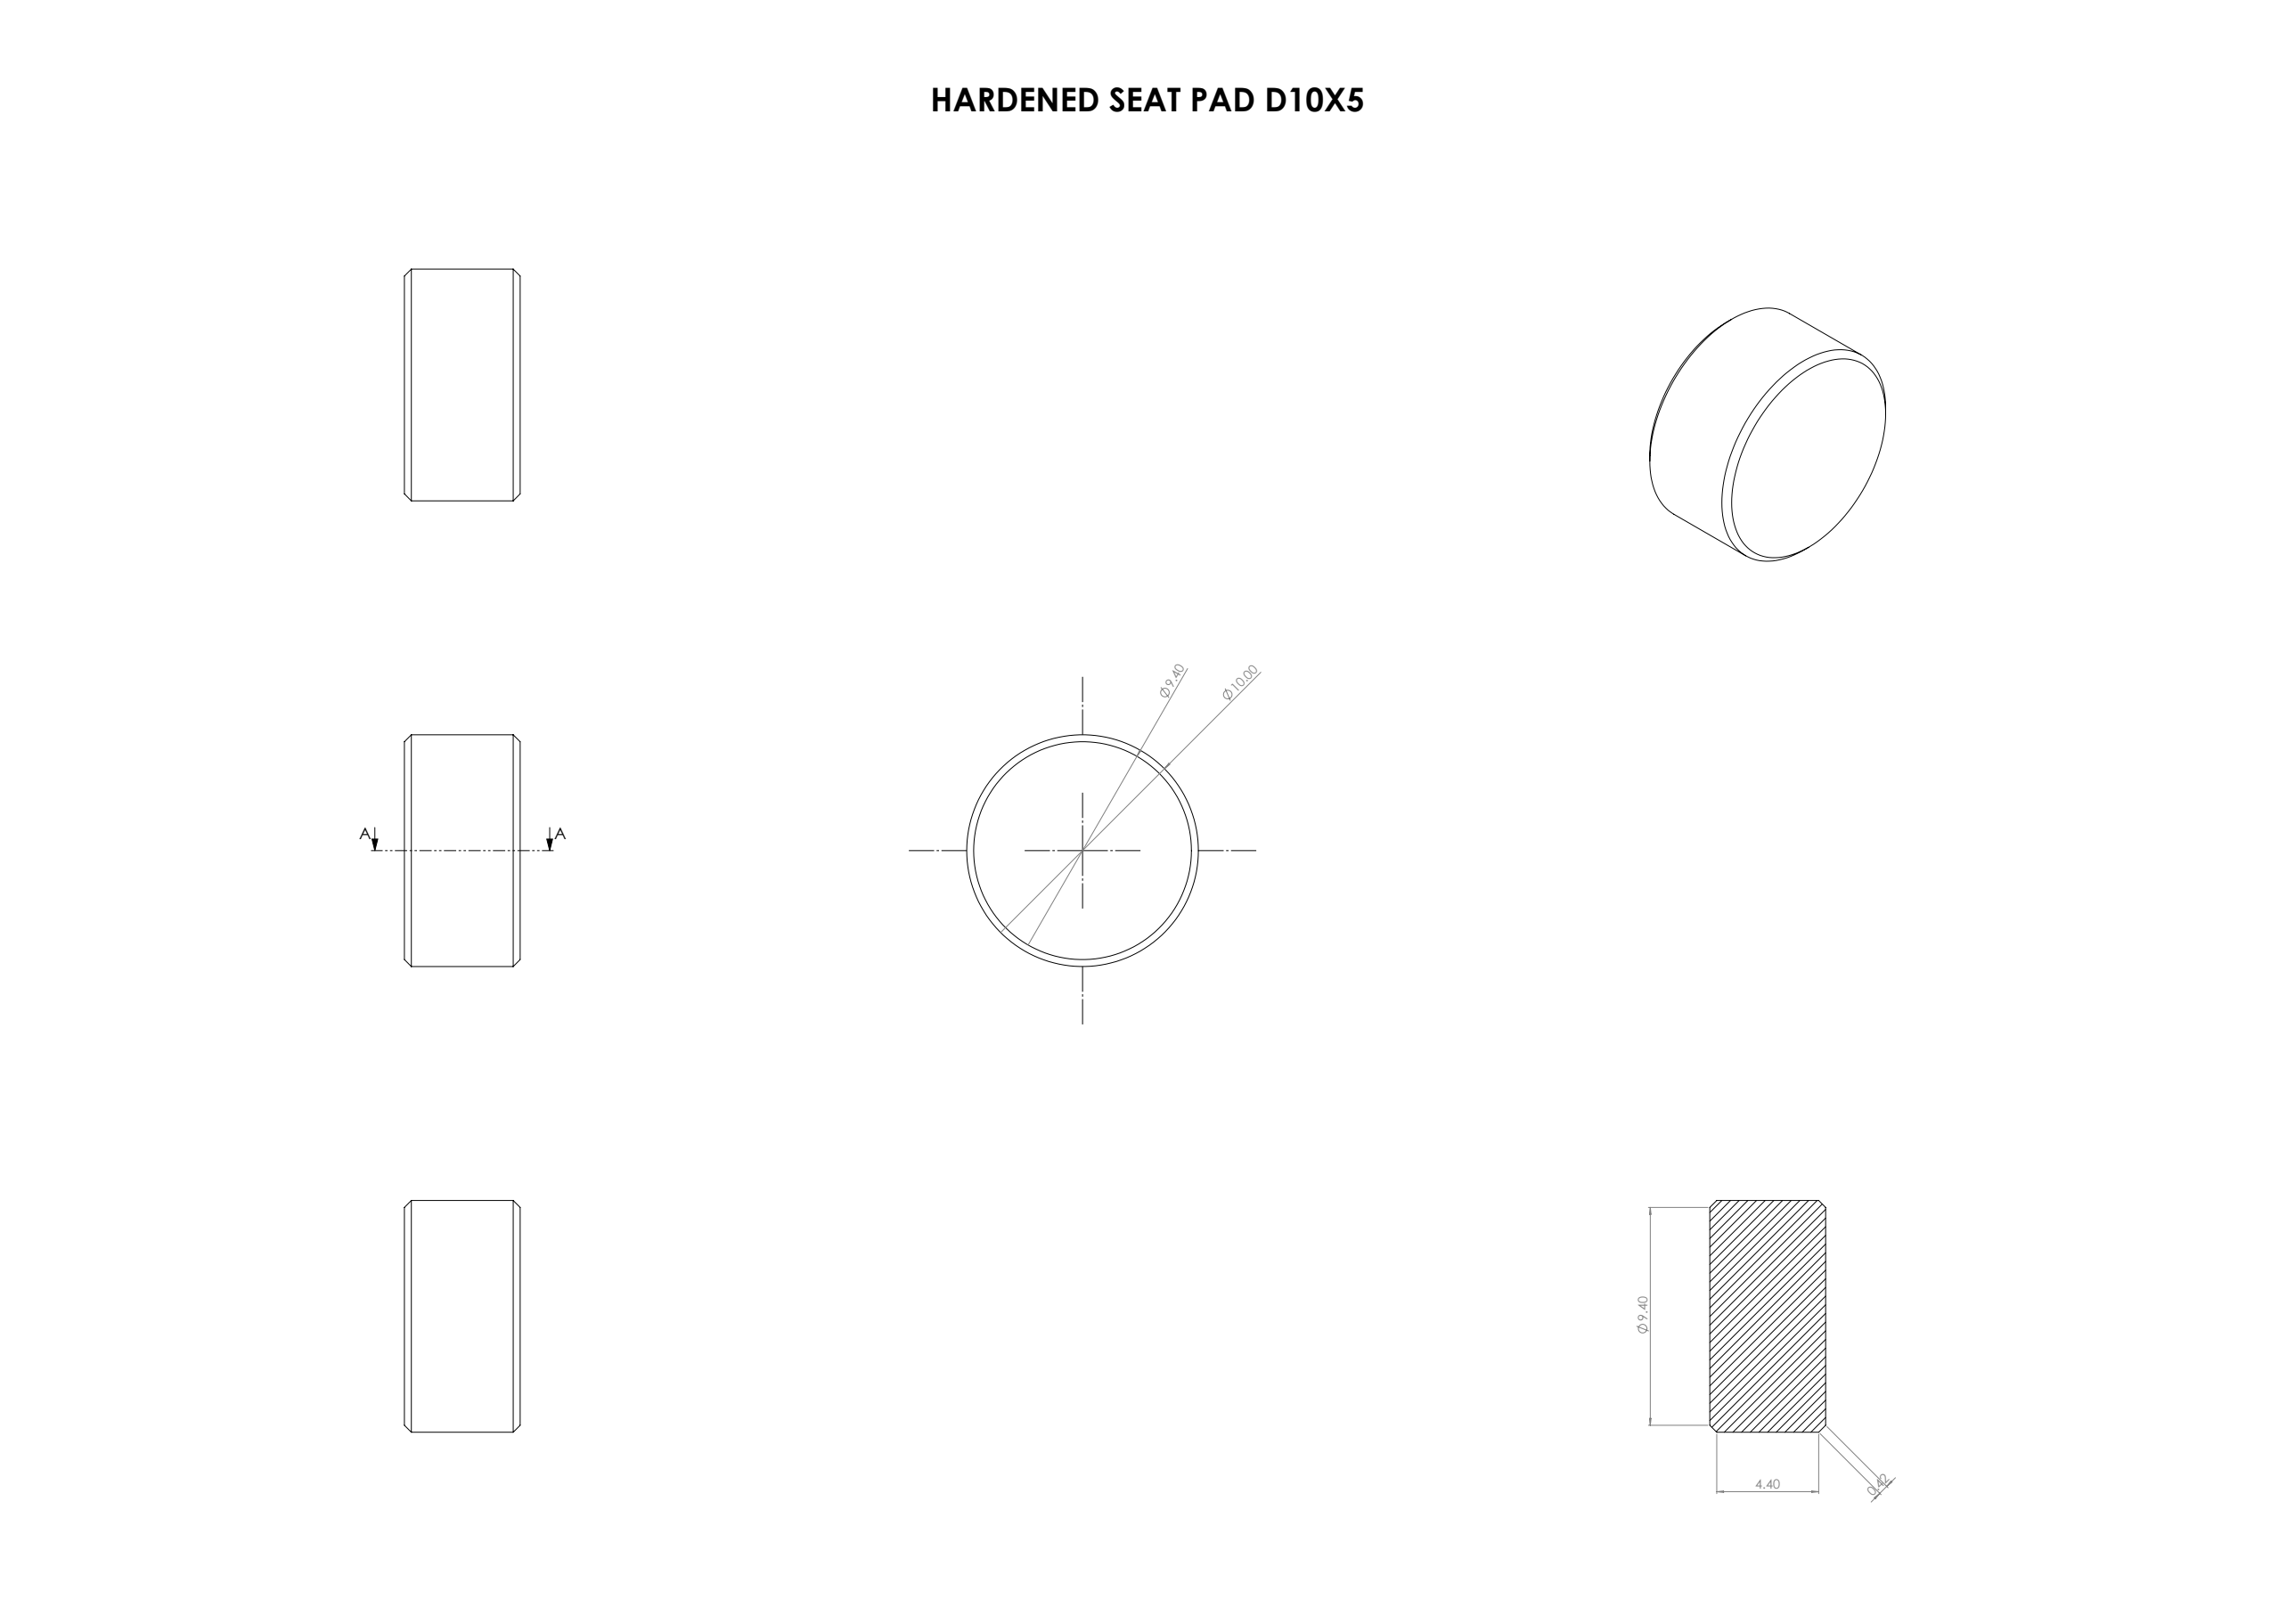
ISO-10303-21;
HEADER;
/* Generated by software containing ST-Developer
 * from STEP Tools, Inc. (www.steptools.com) 
 */

FILE_DESCRIPTION(
/* description */ (''),
/* implementation_level */ '2;1');

FILE_NAME(
/* name */ '10_Hardened_Seat_Pad_D10x5.step',
/* time_stamp */ '2026-10-21T01:56:51-07:00',
/* author */ (''),
/* organization */ (''),
/* preprocessor_version */ 'ST-DEVELOPER v20.2',
/* originating_system */ 'Autodesk Translation Framework v15.15.0.0',
/* authorisation */ '');

FILE_SCHEMA (('AUTOMOTIVE_DESIGN { 1 0 10303 214 3 1 1 }'));
ENDSEC;

DATA;
#10=MECHANICAL_DESIGN_GEOMETRIC_PRESENTATION_REPRESENTATION('',(#278),#82384);
#240=SHAPE_REPRESENTATION_RELATIONSHIP('SRR','None',#82474,#259);
#259=ADVANCED_BREP_SHAPE_REPRESENTATION('',(#297),#82373);
#278=STYLED_ITEM('',(#82617),#297);
#297=MANIFOLD_SOLID_BREP('Body1',#30669);
#575=CYLINDRICAL_SURFACE('',#32083,5.);
#1529=CIRCLE('',#32080,4.7);
#1530=CIRCLE('',#32082,5.);
#1531=CIRCLE('',#32084,5.);
#1532=CIRCLE('',#32086,4.7);
#2035=CONICAL_SURFACE('',#32081,4.85,0.785398163397448);
#2036=CONICAL_SURFACE('',#32085,4.85,0.785398163397448);
#4376=FACE_OUTER_BOUND('',#6334,.T.);
#4377=FACE_OUTER_BOUND('',#6335,.T.);
#4378=FACE_OUTER_BOUND('',#6336,.T.);
#4379=FACE_OUTER_BOUND('',#6337,.T.);
#4380=FACE_OUTER_BOUND('',#6338,.T.);
#6334=EDGE_LOOP('',(#23041));
#6335=EDGE_LOOP('',(#23042,#23043,#23044,#23045));
#6336=EDGE_LOOP('',(#23046,#23047,#23048,#23049));
#6337=EDGE_LOOP('',(#23050,#23051,#23052,#23053));
#6338=EDGE_LOOP('',(#23054));
#8476=LINE('',#48900,#10782);
#8477=LINE('',#48904,#10783);
#8478=LINE('',#48908,#10784);
#10782=VECTOR('',#36893,4.85);
#10783=VECTOR('',#36898,5.);
#10784=VECTOR('',#36903,4.85);
#13181=VERTEX_POINT('',#48895);
#13182=VERTEX_POINT('',#48898);
#13183=VERTEX_POINT('',#48902);
#13184=VERTEX_POINT('',#48906);
#16742=EDGE_CURVE('',#13181,#13181,#1529,.T.);
#16743=EDGE_CURVE('',#13182,#13182,#1530,.T.);
#16744=EDGE_CURVE('',#13182,#13181,#8476,.T.);
#16745=EDGE_CURVE('',#13183,#13183,#1531,.T.);
#16746=EDGE_CURVE('',#13183,#13182,#8477,.T.);
#16747=EDGE_CURVE('',#13184,#13184,#1532,.T.);
#16748=EDGE_CURVE('',#13184,#13183,#8478,.T.);
#23041=ORIENTED_EDGE('',*,*,#16742,.F.);
#23042=ORIENTED_EDGE('',*,*,#16743,.F.);
#23043=ORIENTED_EDGE('',*,*,#16744,.T.);
#23044=ORIENTED_EDGE('',*,*,#16742,.T.);
#23045=ORIENTED_EDGE('',*,*,#16744,.F.);
#23046=ORIENTED_EDGE('',*,*,#16745,.F.);
#23047=ORIENTED_EDGE('',*,*,#16746,.T.);
#23048=ORIENTED_EDGE('',*,*,#16743,.T.);
#23049=ORIENTED_EDGE('',*,*,#16746,.F.);
#23050=ORIENTED_EDGE('',*,*,#16747,.F.);
#23051=ORIENTED_EDGE('',*,*,#16748,.T.);
#23052=ORIENTED_EDGE('',*,*,#16745,.T.);
#23053=ORIENTED_EDGE('',*,*,#16748,.F.);
#23054=ORIENTED_EDGE('',*,*,#16747,.T.);
#28472=PLANE('',#32079);
#28473=PLANE('',#32087);
#29704=ADVANCED_FACE('',(#4376),#28472,.T.);
#29705=ADVANCED_FACE('',(#4377),#2035,.T.);
#29706=ADVANCED_FACE('',(#4378),#575,.T.);
#29707=ADVANCED_FACE('',(#4379),#2036,.T.);
#29708=ADVANCED_FACE('',(#4380),#28473,.T.);
#30669=CLOSED_SHELL('',(#29704,#29705,#29706,#29707,#29708));
#32078=AXIS2_PLACEMENT_3D('',#48893,#36883,#36884);
#32079=AXIS2_PLACEMENT_3D('',#48894,#36885,#36886);
#32080=AXIS2_PLACEMENT_3D('',#48896,#36887,#36888);
#32081=AXIS2_PLACEMENT_3D('',#48897,#36889,#36890);
#32082=AXIS2_PLACEMENT_3D('',#48899,#36891,#36892);
#32083=AXIS2_PLACEMENT_3D('',#48901,#36894,#36895);
#32084=AXIS2_PLACEMENT_3D('',#48903,#36896,#36897);
#32085=AXIS2_PLACEMENT_3D('',#48905,#36899,#36900);
#32086=AXIS2_PLACEMENT_3D('',#48907,#36901,#36902);
#32087=AXIS2_PLACEMENT_3D('',#48909,#36904,#36905);
#36883=DIRECTION('axis',(0.,0.,1.));
#36884=DIRECTION('refdir',(1.,0.,0.));
#36885=DIRECTION('center_axis',(-1.,0.,0.));
#36886=DIRECTION('ref_axis',(0.,0.,1.));
#36887=DIRECTION('center_axis',(1.,0.,0.));
#36888=DIRECTION('ref_axis',(0.,0.,-1.));
#36889=DIRECTION('center_axis',(1.,0.,0.));
#36890=DIRECTION('ref_axis',(0.,1.,0.));
#36891=DIRECTION('center_axis',(1.,0.,0.));
#36892=DIRECTION('ref_axis',(0.,0.,-1.));
#36893=DIRECTION('',(-0.707106781186548,0.707106781186548,8.65956056235493E-17));
#36894=DIRECTION('center_axis',(1.,0.,0.));
#36895=DIRECTION('ref_axis',(0.,1.,0.));
#36896=DIRECTION('center_axis',(1.,0.,0.));
#36897=DIRECTION('ref_axis',(0.,0.,-1.));
#36898=DIRECTION('',(-1.,0.,0.));
#36899=DIRECTION('center_axis',(-1.,0.,0.));
#36900=DIRECTION('ref_axis',(0.,1.,0.));
#36901=DIRECTION('center_axis',(1.,0.,0.));
#36902=DIRECTION('ref_axis',(0.,0.,-1.));
#36903=DIRECTION('',(-0.707106781186548,-0.707106781186547,-8.65956056235493E-17));
#36904=DIRECTION('center_axis',(1.,0.,0.));
#36905=DIRECTION('ref_axis',(0.,0.,-1.));
#48893=CARTESIAN_POINT('',(0.,0.,0.));
#48894=CARTESIAN_POINT('Origin',(-4.5,4.7,0.));
#48895=CARTESIAN_POINT('',(-4.5,-4.7,-5.75583995599256E-16));
#48896=CARTESIAN_POINT('Origin',(-4.5,0.,0.));
#48897=CARTESIAN_POINT('Origin',(-4.35,0.,0.));
#48898=CARTESIAN_POINT('',(-4.2,-5.,-6.12323399573677E-16));
#48899=CARTESIAN_POINT('Origin',(-4.2,0.,0.));
#48900=CARTESIAN_POINT('',(-4.35,-4.85,-5.93953697586466E-16));
#48901=CARTESIAN_POINT('Origin',(-2.,0.,0.));
#48902=CARTESIAN_POINT('',(0.2,-5.,-6.12323399573677E-16));
#48903=CARTESIAN_POINT('Origin',(0.2,0.,0.));
#48904=CARTESIAN_POINT('',(-2.,-5.,-6.12323399573677E-16));
#48905=CARTESIAN_POINT('Origin',(0.35,0.,0.));
#48906=CARTESIAN_POINT('',(0.5,-4.7,-5.75583995599256E-16));
#48907=CARTESIAN_POINT('Origin',(0.5,0.,0.));
#48908=CARTESIAN_POINT('',(0.35,-4.85,-5.93953697586466E-16));
#48909=CARTESIAN_POINT('Origin',(0.5,0.,0.));
#82352=UNCERTAINTY_MEASURE_WITH_UNIT(LENGTH_MEASURE(0.01),#82385,
'DISTANCE_ACCURACY_VALUE',
'Maximum model space distance between geometric entities at asserted c
onnectivities');
#82363=UNCERTAINTY_MEASURE_WITH_UNIT(LENGTH_MEASURE(0.01),#82385,
'DISTANCE_ACCURACY_VALUE',
'Maximum model space distance between geometric entities at asserted c
onnectivities');
#82373=(
GEOMETRIC_REPRESENTATION_CONTEXT(3)
GLOBAL_UNCERTAINTY_ASSIGNED_CONTEXT((#82352))
GLOBAL_UNIT_ASSIGNED_CONTEXT((#82385,#82387,#82388))
REPRESENTATION_CONTEXT('','3D')
);
#82384=(
GEOMETRIC_REPRESENTATION_CONTEXT(3)
GLOBAL_UNCERTAINTY_ASSIGNED_CONTEXT((#82363))
GLOBAL_UNIT_ASSIGNED_CONTEXT((#82385,#82387,#82388))
REPRESENTATION_CONTEXT('','3D')
);
#82385=(
LENGTH_UNIT()
NAMED_UNIT(*)
SI_UNIT(.MILLI.,.METRE.)
);
#82387=(
NAMED_UNIT(*)
PLANE_ANGLE_UNIT()
SI_UNIT($,.RADIAN.)
);
#82388=(
NAMED_UNIT(*)
SI_UNIT($,.STERADIAN.)
SOLID_ANGLE_UNIT()
);
#82398=SHAPE_DEFINITION_REPRESENTATION(#82418,#82474);
#82418=PRODUCT_DEFINITION_SHAPE('',$,#82495);
#82474=SHAPE_REPRESENTATION('',(#32078),#82373);
#82485=PRODUCT_DEFINITION_CONTEXT('part definition',#82547,'design');
#82495=PRODUCT_DEFINITION('2026-10-20-12-38-20-133',
'10_Hardened_Seat_Pad_D10x5',#82515,#82485);
#82515=PRODUCT_DEFINITION_FORMATION('',$,#82558);
#82547=APPLICATION_CONTEXT(
'Core Data for Automotive Mechanical Design Process');
#82548=PRODUCT_CONTEXT('part definition',#82547,'mechanical');
#82558=PRODUCT('2026-10-20-12-38-20-133','10_Hardened_Seat_Pad_D10x5',$,
(#82548));
#82611=COLOUR_RGB('Light Blue',0.38,0.62,0.78);
#82612=FILL_AREA_STYLE_COLOUR('',#82611);
#82613=FILL_AREA_STYLE('',(#82612));
#82614=SURFACE_STYLE_FILL_AREA(#82613);
#82615=SURFACE_SIDE_STYLE('',(#82614));
#82616=SURFACE_STYLE_USAGE(.BOTH.,#82615);
#82617=PRESENTATION_STYLE_ASSIGNMENT((#82616));
ENDSEC;
END-ISO-10303-21;
